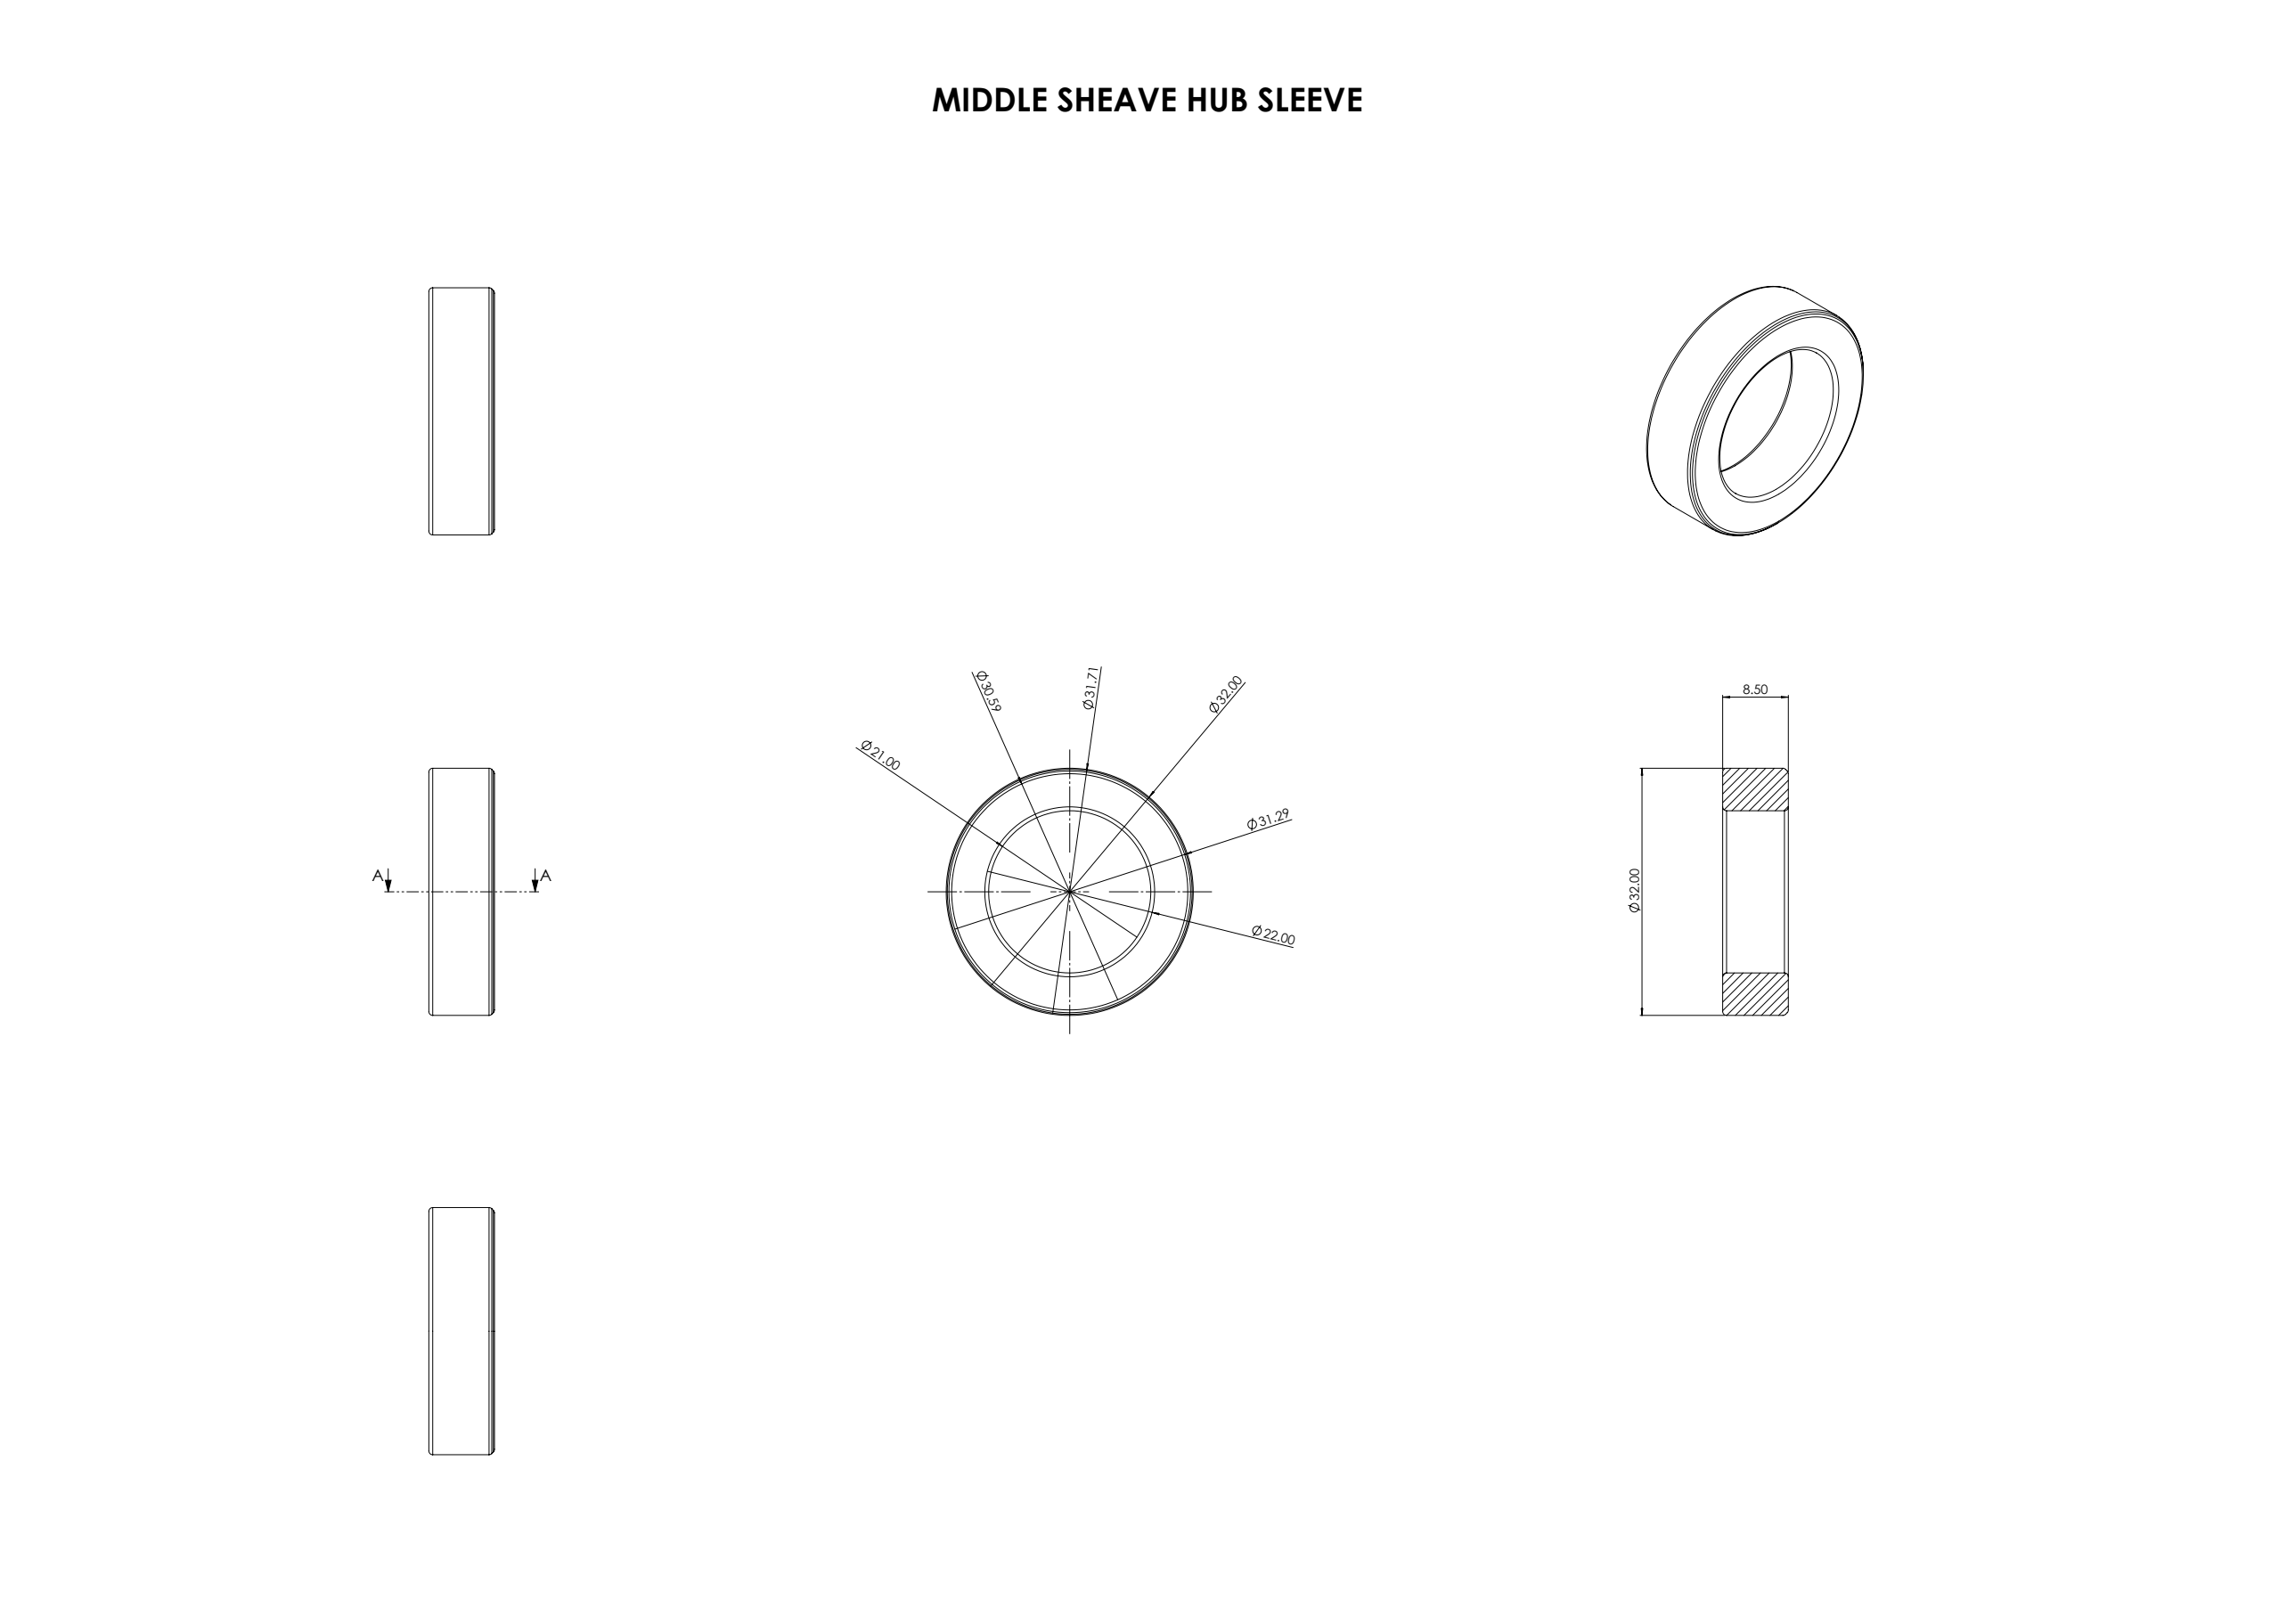
ISO-10303-21;
HEADER;
/* Generated by software containing ST-Developer
 * from STEP Tools, Inc. (www.steptools.com) 
 */

FILE_DESCRIPTION(
/* description */ (''),
/* implementation_level */ '2;1');

FILE_NAME(
/* name */ '06_Middle_Sheave_Hub_Sleeve.step',
/* time_stamp */ '2026-10-24T13:41:11-07:00',
/* author */ (''),
/* organization */ (''),
/* preprocessor_version */ 'ST-DEVELOPER v20.2',
/* originating_system */ 'Autodesk Translation Framework v15.15.0.0',
/* authorisation */ '');

FILE_SCHEMA (('AUTOMOTIVE_DESIGN { 1 0 10303 214 3 1 1 }'));
ENDSEC;

DATA;
#10=MECHANICAL_DESIGN_GEOMETRIC_PRESENTATION_REPRESENTATION('',(#126),#12813);
#96=CONICAL_SURFACE('',#4891,15.75,0.785398163397451);
#106=SHAPE_REPRESENTATION_RELATIONSHIP('SRR','None',#12859,#116);
#116=ADVANCED_BREP_SHAPE_REPRESENTATION('',(#136),#12808);
#126=STYLED_ITEM('',(#12960),#136);
#136=MANIFOLD_SOLID_BREP('Body1',#4389);
#159=FACE_BOUND('',#825,.T.);
#160=FACE_BOUND('',#830,.T.);
#218=PLANE('',#4894);
#219=PLANE('',#4906);
#285=TOROIDAL_SURFACE('',#4886,15.2928932188134,0.5);
#286=TOROIDAL_SURFACE('',#4896,15.5,0.5);
#287=TOROIDAL_SURFACE('',#4903,15.5,0.5);
#288=TOROIDAL_SURFACE('',#4908,11.,0.5);
#289=TOROIDAL_SURFACE('',#4915,11.,0.5);
#534=FACE_OUTER_BOUND('',#822,.T.);
#535=FACE_OUTER_BOUND('',#823,.T.);
#536=FACE_OUTER_BOUND('',#824,.T.);
#537=FACE_OUTER_BOUND('',#826,.T.);
#538=FACE_OUTER_BOUND('',#827,.T.);
#539=FACE_OUTER_BOUND('',#828,.T.);
#540=FACE_OUTER_BOUND('',#829,.T.);
#541=FACE_OUTER_BOUND('',#831,.T.);
#542=FACE_OUTER_BOUND('',#832,.T.);
#543=FACE_OUTER_BOUND('',#833,.T.);
#822=EDGE_LOOP('',(#3785,#3786,#3787,#3788,#3789));
#823=EDGE_LOOP('',(#3790,#3791,#3792,#3793,#3794,#3795));
#824=EDGE_LOOP('',(#3796));
#825=EDGE_LOOP('',(#3797));
#826=EDGE_LOOP('',(#3798,#3799,#3800,#3801,#3802,#3803));
#827=EDGE_LOOP('',(#3804,#3805,#3806,#3807,#3808,#3809));
#828=EDGE_LOOP('',(#3810,#3811,#3812,#3813,#3814));
#829=EDGE_LOOP('',(#3815));
#830=EDGE_LOOP('',(#3816));
#831=EDGE_LOOP('',(#3817,#3818,#3819,#3820,#3821));
#832=EDGE_LOOP('',(#3822,#3823,#3824,#3825,#3826,#3827));
#833=EDGE_LOOP('',(#3828,#3829,#3830,#3831,#3832));
#1082=CIRCLE('',#4887,15.2928932188134);
#1083=CIRCLE('',#4888,0.5);
#1084=CIRCLE('',#4889,15.6464466094067);
#1085=CIRCLE('',#4890,15.6464466094067);
#1086=CIRCLE('',#4892,15.8535533905933);
#1087=CIRCLE('',#4893,15.8535533905933);
#1088=CIRCLE('',#4895,11.);
#1089=CIRCLE('',#4897,0.5);
#1090=CIRCLE('',#4898,16.);
#1091=CIRCLE('',#4899,16.);
#1092=CIRCLE('',#4901,16.);
#1093=CIRCLE('',#4902,16.);
#1094=CIRCLE('',#4904,0.5);
#1095=CIRCLE('',#4905,15.5);
#1096=CIRCLE('',#4907,11.);
#1097=CIRCLE('',#4909,0.5);
#1098=CIRCLE('',#4910,10.5);
#1099=CIRCLE('',#4911,10.5);
#1100=CIRCLE('',#4913,10.5);
#1101=CIRCLE('',#4914,10.5);
#1102=CIRCLE('',#4916,0.5);
#1272=LINE('',#12529,#1502);
#1273=LINE('',#12544,#1503);
#1274=LINE('',#12566,#1504);
#1502=VECTOR('',#5927,15.75);
#1503=VECTOR('',#5946,16.);
#1504=VECTOR('',#5975,10.5);
#2064=VERTEX_POINT('',#12520);
#2065=VERTEX_POINT('',#12522);
#2066=VERTEX_POINT('',#12524);
#2067=VERTEX_POINT('',#12528);
#2068=VERTEX_POINT('',#12530);
#2069=VERTEX_POINT('',#12534);
#2070=VERTEX_POINT('',#12537);
#2071=VERTEX_POINT('',#12539);
#2072=VERTEX_POINT('',#12543);
#2073=VERTEX_POINT('',#12545);
#2074=VERTEX_POINT('',#12549);
#2075=VERTEX_POINT('',#12553);
#2076=VERTEX_POINT('',#12556);
#2077=VERTEX_POINT('',#12558);
#2078=VERTEX_POINT('',#12562);
#2079=VERTEX_POINT('',#12563);
#2645=EDGE_CURVE('',#2064,#2064,#1082,.T.);
#2646=EDGE_CURVE('',#2064,#2065,#1083,.T.);
#2647=EDGE_CURVE('',#2065,#2066,#1084,.T.);
#2648=EDGE_CURVE('',#2066,#2065,#1085,.T.);
#2649=EDGE_CURVE('',#2066,#2067,#1272,.T.);
#2650=EDGE_CURVE('',#2068,#2067,#1086,.T.);
#2651=EDGE_CURVE('',#2067,#2068,#1087,.T.);
#2652=EDGE_CURVE('',#2069,#2069,#1088,.T.);
#2653=EDGE_CURVE('',#2068,#2070,#1089,.T.);
#2654=EDGE_CURVE('',#2070,#2071,#1090,.T.);
#2655=EDGE_CURVE('',#2071,#2070,#1091,.T.);
#2656=EDGE_CURVE('',#2071,#2072,#1273,.T.);
#2657=EDGE_CURVE('',#2073,#2072,#1092,.T.);
#2658=EDGE_CURVE('',#2072,#2073,#1093,.T.);
#2659=EDGE_CURVE('',#2073,#2074,#1094,.T.);
#2660=EDGE_CURVE('',#2074,#2074,#1095,.T.);
#2661=EDGE_CURVE('',#2075,#2075,#1096,.T.);
#2662=EDGE_CURVE('',#2075,#2076,#1097,.T.);
#2663=EDGE_CURVE('',#2076,#2077,#1098,.T.);
#2664=EDGE_CURVE('',#2077,#2076,#1099,.T.);
#2665=EDGE_CURVE('',#2078,#2079,#1100,.T.);
#2666=EDGE_CURVE('',#2079,#2078,#1101,.T.);
#2667=EDGE_CURVE('',#2079,#2077,#1274,.T.);
#2668=EDGE_CURVE('',#2078,#2069,#1102,.T.);
#3785=ORIENTED_EDGE('',*,*,#2645,.T.);
#3786=ORIENTED_EDGE('',*,*,#2646,.T.);
#3787=ORIENTED_EDGE('',*,*,#2647,.T.);
#3788=ORIENTED_EDGE('',*,*,#2648,.T.);
#3789=ORIENTED_EDGE('',*,*,#2646,.F.);
#3790=ORIENTED_EDGE('',*,*,#2648,.F.);
#3791=ORIENTED_EDGE('',*,*,#2649,.T.);
#3792=ORIENTED_EDGE('',*,*,#2650,.F.);
#3793=ORIENTED_EDGE('',*,*,#2651,.F.);
#3794=ORIENTED_EDGE('',*,*,#2649,.F.);
#3795=ORIENTED_EDGE('',*,*,#2647,.F.);
#3796=ORIENTED_EDGE('',*,*,#2645,.F.);
#3797=ORIENTED_EDGE('',*,*,#2652,.F.);
#3798=ORIENTED_EDGE('',*,*,#2650,.T.);
#3799=ORIENTED_EDGE('',*,*,#2651,.T.);
#3800=ORIENTED_EDGE('',*,*,#2653,.T.);
#3801=ORIENTED_EDGE('',*,*,#2654,.T.);
#3802=ORIENTED_EDGE('',*,*,#2655,.T.);
#3803=ORIENTED_EDGE('',*,*,#2653,.F.);
#3804=ORIENTED_EDGE('',*,*,#2655,.F.);
#3805=ORIENTED_EDGE('',*,*,#2656,.T.);
#3806=ORIENTED_EDGE('',*,*,#2657,.F.);
#3807=ORIENTED_EDGE('',*,*,#2658,.F.);
#3808=ORIENTED_EDGE('',*,*,#2656,.F.);
#3809=ORIENTED_EDGE('',*,*,#2654,.F.);
#3810=ORIENTED_EDGE('',*,*,#2657,.T.);
#3811=ORIENTED_EDGE('',*,*,#2658,.T.);
#3812=ORIENTED_EDGE('',*,*,#2659,.T.);
#3813=ORIENTED_EDGE('',*,*,#2660,.T.);
#3814=ORIENTED_EDGE('',*,*,#2659,.F.);
#3815=ORIENTED_EDGE('',*,*,#2660,.F.);
#3816=ORIENTED_EDGE('',*,*,#2661,.F.);
#3817=ORIENTED_EDGE('',*,*,#2661,.T.);
#3818=ORIENTED_EDGE('',*,*,#2662,.T.);
#3819=ORIENTED_EDGE('',*,*,#2663,.T.);
#3820=ORIENTED_EDGE('',*,*,#2664,.T.);
#3821=ORIENTED_EDGE('',*,*,#2662,.F.);
#3822=ORIENTED_EDGE('',*,*,#2665,.F.);
#3823=ORIENTED_EDGE('',*,*,#2666,.F.);
#3824=ORIENTED_EDGE('',*,*,#2667,.T.);
#3825=ORIENTED_EDGE('',*,*,#2663,.F.);
#3826=ORIENTED_EDGE('',*,*,#2664,.F.);
#3827=ORIENTED_EDGE('',*,*,#2667,.F.);
#3828=ORIENTED_EDGE('',*,*,#2665,.T.);
#3829=ORIENTED_EDGE('',*,*,#2666,.T.);
#3830=ORIENTED_EDGE('',*,*,#2668,.T.);
#3831=ORIENTED_EDGE('',*,*,#2652,.T.);
#3832=ORIENTED_EDGE('',*,*,#2668,.F.);
#4104=CYLINDRICAL_SURFACE('',#4900,16.);
#4105=CYLINDRICAL_SURFACE('',#4912,10.5);
#4324=ADVANCED_FACE('',(#534),#285,.T.);
#4325=ADVANCED_FACE('',(#535),#96,.T.);
#4326=ADVANCED_FACE('',(#536,#159),#218,.T.);
#4327=ADVANCED_FACE('',(#537),#286,.T.);
#4328=ADVANCED_FACE('',(#538),#4104,.T.);
#4329=ADVANCED_FACE('',(#539),#287,.T.);
#4330=ADVANCED_FACE('',(#540,#160),#219,.T.);
#4331=ADVANCED_FACE('',(#541),#288,.T.);
#4332=ADVANCED_FACE('',(#542),#4105,.F.);
#4333=ADVANCED_FACE('',(#543),#289,.T.);
#4389=CLOSED_SHELL('',(#4324,#4325,#4326,#4327,#4328,#4329,#4330,#4331,
#4332,#4333));
#4885=AXIS2_PLACEMENT_3D('',#12518,#5913,#5914);
#4886=AXIS2_PLACEMENT_3D('',#12519,#5915,#5916);
#4887=AXIS2_PLACEMENT_3D('',#12521,#5917,#5918);
#4888=AXIS2_PLACEMENT_3D('',#12523,#5919,#5920);
#4889=AXIS2_PLACEMENT_3D('',#12525,#5921,#5922);
#4890=AXIS2_PLACEMENT_3D('',#12526,#5923,#5924);
#4891=AXIS2_PLACEMENT_3D('',#12527,#5925,#5926);
#4892=AXIS2_PLACEMENT_3D('',#12531,#5928,#5929);
#4893=AXIS2_PLACEMENT_3D('',#12532,#5930,#5931);
#4894=AXIS2_PLACEMENT_3D('',#12533,#5932,#5933);
#4895=AXIS2_PLACEMENT_3D('',#12535,#5934,#5935);
#4896=AXIS2_PLACEMENT_3D('',#12536,#5936,#5937);
#4897=AXIS2_PLACEMENT_3D('',#12538,#5938,#5939);
#4898=AXIS2_PLACEMENT_3D('',#12540,#5940,#5941);
#4899=AXIS2_PLACEMENT_3D('',#12541,#5942,#5943);
#4900=AXIS2_PLACEMENT_3D('',#12542,#5944,#5945);
#4901=AXIS2_PLACEMENT_3D('',#12546,#5947,#5948);
#4902=AXIS2_PLACEMENT_3D('',#12547,#5949,#5950);
#4903=AXIS2_PLACEMENT_3D('',#12548,#5951,#5952);
#4904=AXIS2_PLACEMENT_3D('',#12550,#5953,#5954);
#4905=AXIS2_PLACEMENT_3D('',#12551,#5955,#5956);
#4906=AXIS2_PLACEMENT_3D('',#12552,#5957,#5958);
#4907=AXIS2_PLACEMENT_3D('',#12554,#5959,#5960);
#4908=AXIS2_PLACEMENT_3D('',#12555,#5961,#5962);
#4909=AXIS2_PLACEMENT_3D('',#12557,#5963,#5964);
#4910=AXIS2_PLACEMENT_3D('',#12559,#5965,#5966);
#4911=AXIS2_PLACEMENT_3D('',#12560,#5967,#5968);
#4912=AXIS2_PLACEMENT_3D('',#12561,#5969,#5970);
#4913=AXIS2_PLACEMENT_3D('',#12564,#5971,#5972);
#4914=AXIS2_PLACEMENT_3D('',#12565,#5973,#5974);
#4915=AXIS2_PLACEMENT_3D('',#12567,#5976,#5977);
#4916=AXIS2_PLACEMENT_3D('',#12568,#5978,#5979);
#5913=DIRECTION('axis',(0.,0.,1.));
#5914=DIRECTION('refdir',(1.,0.,0.));
#5915=DIRECTION('center_axis',(1.,0.,0.));
#5916=DIRECTION('ref_axis',(0.,0.,-1.));
#5917=DIRECTION('center_axis',(-1.,0.,0.));
#5918=DIRECTION('ref_axis',(0.,-1.,1.83697019872103E-16));
#5919=DIRECTION('center_axis',(0.,-1.,-1.22464679914735E-16));
#5920=DIRECTION('ref_axis',(0.,-1.22464679914735E-16,1.));
#5921=DIRECTION('center_axis',(1.,0.,0.));
#5922=DIRECTION('ref_axis',(0.,-1.,3.06161699786838E-17));
#5923=DIRECTION('center_axis',(1.,0.,0.));
#5924=DIRECTION('ref_axis',(0.,-1.,3.06161699786838E-17));
#5925=DIRECTION('center_axis',(-1.,0.,0.));
#5926=DIRECTION('ref_axis',(0.,1.,0.));
#5927=DIRECTION('',(-0.707106781186546,-0.707106781186549,-8.65956056235495E-17));
#5928=DIRECTION('center_axis',(-1.,0.,0.));
#5929=DIRECTION('ref_axis',(0.,-1.,3.06161699786838E-17));
#5930=DIRECTION('center_axis',(-1.,0.,0.));
#5931=DIRECTION('ref_axis',(0.,-1.,3.06161699786838E-17));
#5932=DIRECTION('center_axis',(1.,0.,0.));
#5933=DIRECTION('ref_axis',(0.,0.,-1.));
#5934=DIRECTION('center_axis',(1.,0.,0.));
#5935=DIRECTION('ref_axis',(0.,-1.,1.83697019872103E-16));
#5936=DIRECTION('center_axis',(1.,0.,0.));
#5937=DIRECTION('ref_axis',(0.,0.,-1.));
#5938=DIRECTION('center_axis',(0.,-1.,-1.22464679914735E-16));
#5939=DIRECTION('ref_axis',(0.,-1.22464679914735E-16,1.));
#5940=DIRECTION('center_axis',(1.,0.,0.));
#5941=DIRECTION('ref_axis',(0.,-1.,1.83697019872103E-16));
#5942=DIRECTION('center_axis',(1.,0.,0.));
#5943=DIRECTION('ref_axis',(0.,-1.,1.83697019872103E-16));
#5944=DIRECTION('center_axis',(1.,0.,0.));
#5945=DIRECTION('ref_axis',(0.,1.,0.));
#5946=DIRECTION('',(-1.,0.,0.));
#5947=DIRECTION('center_axis',(-1.,0.,0.));
#5948=DIRECTION('ref_axis',(0.,-1.,1.83697019872103E-16));
#5949=DIRECTION('center_axis',(-1.,0.,0.));
#5950=DIRECTION('ref_axis',(0.,-1.,1.83697019872103E-16));
#5951=DIRECTION('center_axis',(1.,0.,0.));
#5952=DIRECTION('ref_axis',(0.,0.,-1.));
#5953=DIRECTION('center_axis',(0.,-1.,-1.22464679914735E-16));
#5954=DIRECTION('ref_axis',(0.,-1.22464679914735E-16,1.));
#5955=DIRECTION('center_axis',(1.,0.,0.));
#5956=DIRECTION('ref_axis',(0.,-1.,1.83697019872103E-16));
#5957=DIRECTION('center_axis',(-1.,0.,0.));
#5958=DIRECTION('ref_axis',(0.,0.,1.));
#5959=DIRECTION('center_axis',(-1.,0.,0.));
#5960=DIRECTION('ref_axis',(0.,-1.,1.83697019872103E-16));
#5961=DIRECTION('center_axis',(1.,0.,0.));
#5962=DIRECTION('ref_axis',(0.,0.,-1.));
#5963=DIRECTION('center_axis',(0.,-1.,-1.22464679914735E-16));
#5964=DIRECTION('ref_axis',(0.,-1.22464679914735E-16,1.));
#5965=DIRECTION('center_axis',(1.,0.,0.));
#5966=DIRECTION('ref_axis',(0.,-1.,1.83697019872103E-16));
#5967=DIRECTION('center_axis',(1.,0.,0.));
#5968=DIRECTION('ref_axis',(0.,-1.,1.83697019872103E-16));
#5969=DIRECTION('center_axis',(1.,0.,0.));
#5970=DIRECTION('ref_axis',(0.,1.,0.));
#5971=DIRECTION('center_axis',(-1.,0.,0.));
#5972=DIRECTION('ref_axis',(0.,-1.,1.83697019872103E-16));
#5973=DIRECTION('center_axis',(-1.,0.,0.));
#5974=DIRECTION('ref_axis',(0.,-1.,1.83697019872103E-16));
#5975=DIRECTION('',(-1.,0.,0.));
#5976=DIRECTION('center_axis',(1.,0.,0.));
#5977=DIRECTION('ref_axis',(0.,0.,-1.));
#5978=DIRECTION('center_axis',(0.,-1.,-1.22464679914735E-16));
#5979=DIRECTION('ref_axis',(0.,-1.22464679914735E-16,1.));
#12518=CARTESIAN_POINT('',(0.,0.,0.));
#12519=CARTESIAN_POINT('Origin',(42.,0.,0.));
#12520=CARTESIAN_POINT('',(42.5,-1.87283927301222E-15,15.2928932188134));
#12521=CARTESIAN_POINT('Origin',(42.5,0.,0.));
#12522=CARTESIAN_POINT('',(42.3535533905933,-1.91613707582399E-15,15.6464466094067));
#12523=CARTESIAN_POINT('Origin',(42.,-1.87283927301222E-15,15.2928932188134));
#12524=CARTESIAN_POINT('',(42.3535533905933,-15.6464466094067,-1.91613707582399E-15));
#12525=CARTESIAN_POINT('Origin',(42.3535533905933,0.,-2.39517134477999E-15));
#12526=CARTESIAN_POINT('Origin',(42.3535533905933,0.,-2.39517134477999E-15));
#12527=CARTESIAN_POINT('Origin',(42.25,0.,0.));
#12528=CARTESIAN_POINT('',(42.1464466094067,-15.8535533905933,-1.94150034149017E-15));
#12529=CARTESIAN_POINT('',(42.25,-15.75,-1.92881870865708E-15));
#12530=CARTESIAN_POINT('',(42.1464466094067,-1.94150034149017E-15,15.8535533905933));
#12531=CARTESIAN_POINT('Origin',(42.1464466094067,0.,-2.42687542686271E-15));
#12532=CARTESIAN_POINT('Origin',(42.1464466094067,0.,-2.42687542686271E-15));
#12533=CARTESIAN_POINT('Origin',(42.5,10.5,0.));
#12534=CARTESIAN_POINT('',(42.5,-1.34711147906209E-15,11.));
#12535=CARTESIAN_POINT('Origin',(42.5,0.,0.));
#12536=CARTESIAN_POINT('Origin',(41.7928932188135,0.,0.));
#12537=CARTESIAN_POINT('',(41.7928932188135,-1.95943487863577E-15,16.));
#12538=CARTESIAN_POINT('Origin',(41.7928932188135,-1.8982025386784E-15,
15.5));
#12539=CARTESIAN_POINT('',(41.7928932188135,-16.,-1.95943487863577E-15));
#12540=CARTESIAN_POINT('Origin',(41.7928932188135,0.,0.));
#12541=CARTESIAN_POINT('Origin',(41.7928932188135,0.,0.));
#12542=CARTESIAN_POINT('Origin',(38.,0.,0.));
#12543=CARTESIAN_POINT('',(34.5,-16.,-1.95943487863577E-15));
#12544=CARTESIAN_POINT('',(38.,-16.,-1.95943487863577E-15));
#12545=CARTESIAN_POINT('',(34.5,-1.95943487863577E-15,16.));
#12546=CARTESIAN_POINT('Origin',(34.5,0.,0.));
#12547=CARTESIAN_POINT('Origin',(34.5,0.,0.));
#12548=CARTESIAN_POINT('Origin',(34.5,0.,0.));
#12549=CARTESIAN_POINT('',(34.,-1.8982025386784E-15,15.5));
#12550=CARTESIAN_POINT('Origin',(34.5,-1.8982025386784E-15,15.5));
#12551=CARTESIAN_POINT('Origin',(34.,0.,0.));
#12552=CARTESIAN_POINT('Origin',(34.,16.,0.));
#12553=CARTESIAN_POINT('',(34.,-1.34711147906209E-15,11.));
#12554=CARTESIAN_POINT('Origin',(34.,0.,0.));
#12555=CARTESIAN_POINT('Origin',(34.5,0.,0.));
#12556=CARTESIAN_POINT('',(34.5,-1.28587913910472E-15,10.5));
#12557=CARTESIAN_POINT('Origin',(34.5,-1.34711147906209E-15,11.));
#12558=CARTESIAN_POINT('',(34.5,-10.5,-1.28587913910472E-15));
#12559=CARTESIAN_POINT('Origin',(34.5,0.,0.));
#12560=CARTESIAN_POINT('Origin',(34.5,0.,0.));
#12561=CARTESIAN_POINT('Origin',(38.25,0.,0.));
#12562=CARTESIAN_POINT('',(42.,-1.28587913910472E-15,10.5));
#12563=CARTESIAN_POINT('',(42.,-10.5,-1.28587913910472E-15));
#12564=CARTESIAN_POINT('Origin',(42.,0.,0.));
#12565=CARTESIAN_POINT('Origin',(42.,0.,0.));
#12566=CARTESIAN_POINT('',(38.25,-10.5,-1.28587913910472E-15));
#12567=CARTESIAN_POINT('Origin',(42.,0.,0.));
#12568=CARTESIAN_POINT('Origin',(42.,-1.34711147906209E-15,11.));
#12796=UNCERTAINTY_MEASURE_WITH_UNIT(LENGTH_MEASURE(0.01),#12814,
'DISTANCE_ACCURACY_VALUE',
'Maximum model space distance between geometric entities at asserted c
onnectivities');
#12801=UNCERTAINTY_MEASURE_WITH_UNIT(LENGTH_MEASURE(0.01),#12814,
'DISTANCE_ACCURACY_VALUE',
'Maximum model space distance between geometric entities at asserted c
onnectivities');
#12808=(
GEOMETRIC_REPRESENTATION_CONTEXT(3)
GLOBAL_UNCERTAINTY_ASSIGNED_CONTEXT((#12796))
GLOBAL_UNIT_ASSIGNED_CONTEXT((#12814,#12816,#12817))
REPRESENTATION_CONTEXT('','3D')
);
#12813=(
GEOMETRIC_REPRESENTATION_CONTEXT(3)
GLOBAL_UNCERTAINTY_ASSIGNED_CONTEXT((#12801))
GLOBAL_UNIT_ASSIGNED_CONTEXT((#12814,#12816,#12817))
REPRESENTATION_CONTEXT('','3D')
);
#12814=(
LENGTH_UNIT()
NAMED_UNIT(*)
SI_UNIT(.MILLI.,.METRE.)
);
#12816=(
NAMED_UNIT(*)
PLANE_ANGLE_UNIT()
SI_UNIT($,.RADIAN.)
);
#12817=(
NAMED_UNIT(*)
SI_UNIT($,.STERADIAN.)
SOLID_ANGLE_UNIT()
);
#12824=SHAPE_DEFINITION_REPRESENTATION(#12835,#12859);
#12835=PRODUCT_DEFINITION_SHAPE('',$,#12871);
#12859=SHAPE_REPRESENTATION('',(#4885),#12808);
#12864=PRODUCT_DEFINITION_CONTEXT('part definition',#12899,'design');
#12871=PRODUCT_DEFINITION('2026-10-11-12-17-36-060',
'06_Middle_Sheave_Hub_Sleeve',#12882,#12864);
#12882=PRODUCT_DEFINITION_FORMATION('',$,#12907);
#12899=APPLICATION_CONTEXT(
'Core Data for Automotive Mechanical Design Process');
#12900=PRODUCT_CONTEXT('part definition',#12899,'mechanical');
#12907=PRODUCT('2026-10-11-12-17-36-060','06_Middle_Sheave_Hub_Sleeve',
$,(#12900));
#12954=COLOUR_RGB('Light Blue',0.38,0.62,0.78);
#12955=FILL_AREA_STYLE_COLOUR('',#12954);
#12956=FILL_AREA_STYLE('',(#12955));
#12957=SURFACE_STYLE_FILL_AREA(#12956);
#12958=SURFACE_SIDE_STYLE('',(#12957));
#12959=SURFACE_STYLE_USAGE(.BOTH.,#12958);
#12960=PRESENTATION_STYLE_ASSIGNMENT((#12959));
ENDSEC;
END-ISO-10303-21;
